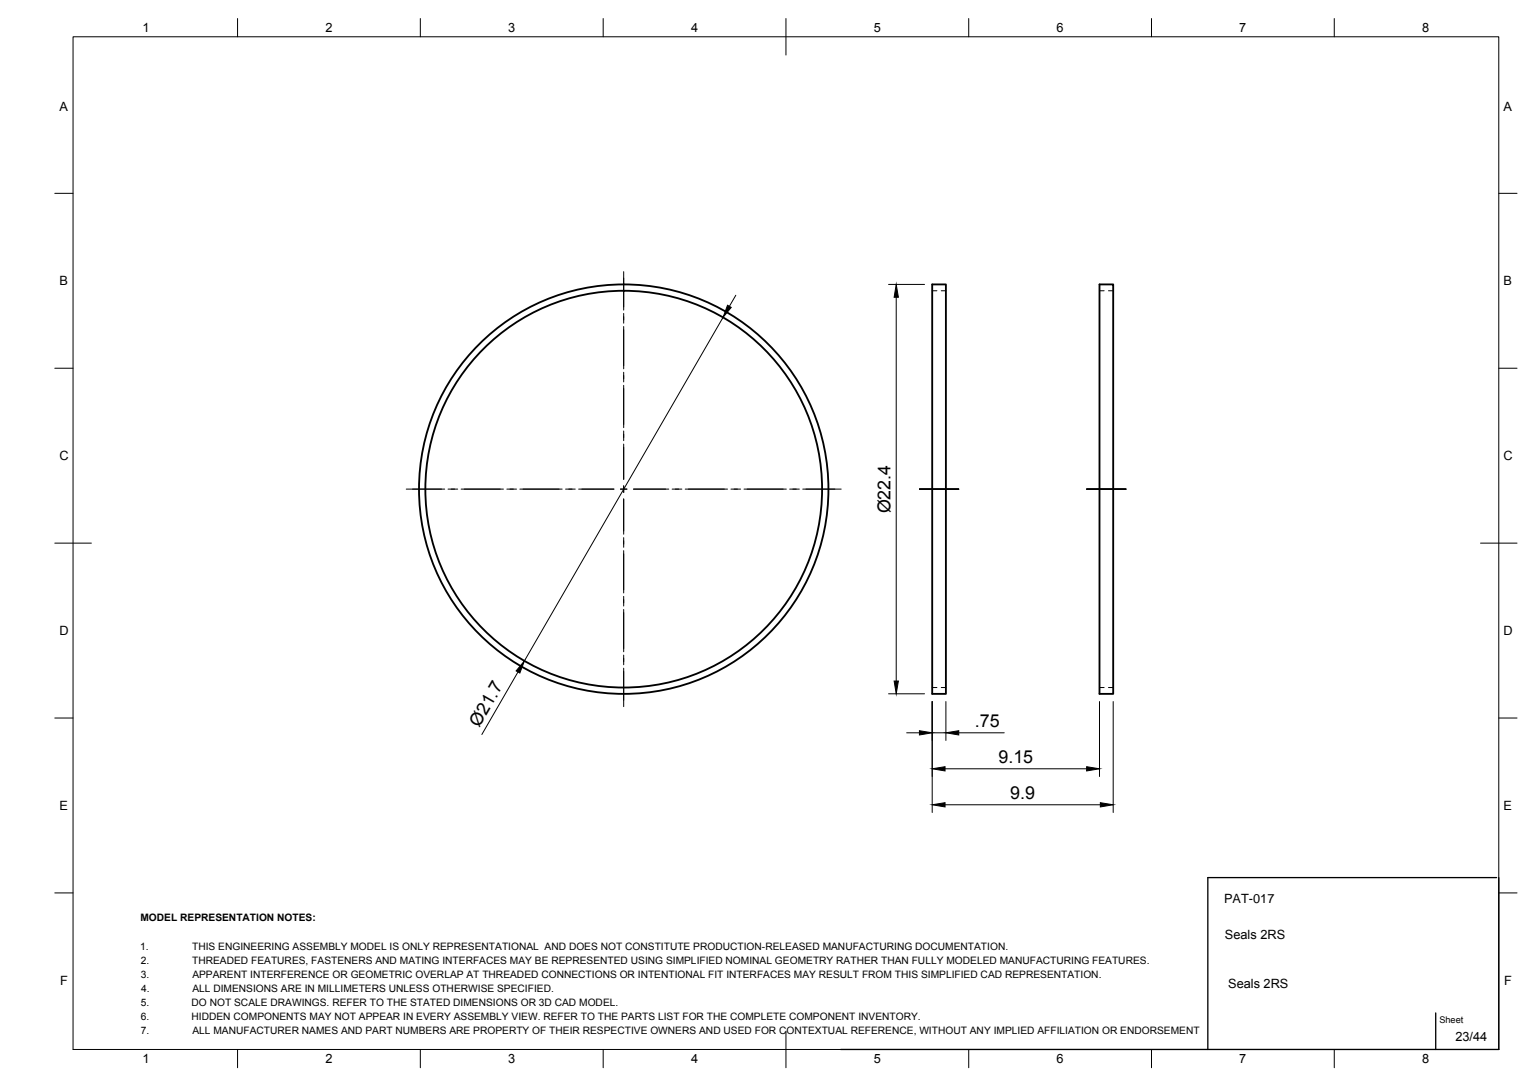
ISO-10303-21;
HEADER;
/* Generated by software containing ST-Developer
 * from STEP Tools, Inc. (www.steptools.com) 
 */

FILE_DESCRIPTION(
/* description */ ('Cam-and-follower valve demonstrator'),
/* implementation_level */ '2;1');

FILE_NAME(
/* name */ 'Seals 2RS.step',
/* time_stamp */ '2026-10-28T03:25:17-07:00',
/* author */ (''),
/* organization */ (''),
/* preprocessor_version */ 'ST-DEVELOPER v20.2',
/* originating_system */ 'Autodesk Translation Framework v15.17.0.0',
/* authorisation */ '');

FILE_SCHEMA (('AUTOMOTIVE_DESIGN { 1 0 10303 214 3 1 1 }'));
ENDSEC;

DATA;
#10=MECHANICAL_DESIGN_GEOMETRIC_PRESENTATION_REPRESENTATION('',(#434,#435),#12896);
#356=SHAPE_REPRESENTATION_RELATIONSHIP('SRR','None',#13073,#392);
#392=ADVANCED_BREP_SHAPE_REPRESENTATION('',(#477,#478),#12873);
#434=STYLED_ITEM('',(#13330),#477);
#435=STYLED_ITEM('',(#13330),#478);
#477=MANIFOLD_SOLID_BREP('Body1',#6201);
#478=MANIFOLD_SOLID_BREP('Body2',#6202);
#609=FACE_BOUND('',#1765,.T.);
#610=FACE_BOUND('',#1768,.T.);
#611=FACE_BOUND('',#1771,.T.);
#612=FACE_BOUND('',#1774,.T.);
#852=CIRCLE('',#7022,1.119765);
#853=CIRCLE('',#7023,1.085235);
#854=CIRCLE('',#7025,1.119765);
#855=CIRCLE('',#7027,1.085235);
#856=CIRCLE('',#7030,1.119765);
#857=CIRCLE('',#7031,1.085235);
#858=CIRCLE('',#7033,1.119765);
#859=CIRCLE('',#7035,1.085235);
#1046=CYLINDRICAL_SURFACE('',#7024,1.119765);
#1047=CYLINDRICAL_SURFACE('',#7028,1.085235);
#1048=CYLINDRICAL_SURFACE('',#7032,1.119765);
#1049=CYLINDRICAL_SURFACE('',#7036,1.085235);
#1282=FACE_OUTER_BOUND('',#1764,.T.);
#1283=FACE_OUTER_BOUND('',#1766,.T.);
#1284=FACE_OUTER_BOUND('',#1767,.T.);
#1285=FACE_OUTER_BOUND('',#1769,.T.);
#1286=FACE_OUTER_BOUND('',#1770,.T.);
#1287=FACE_OUTER_BOUND('',#1772,.T.);
#1288=FACE_OUTER_BOUND('',#1773,.T.);
#1289=FACE_OUTER_BOUND('',#1775,.T.);
#1764=EDGE_LOOP('',(#4929));
#1765=EDGE_LOOP('',(#4930));
#1766=EDGE_LOOP('',(#4931,#4932,#4933,#4934));
#1767=EDGE_LOOP('',(#4935));
#1768=EDGE_LOOP('',(#4936));
#1769=EDGE_LOOP('',(#4937,#4938,#4939,#4940));
#1770=EDGE_LOOP('',(#4941));
#1771=EDGE_LOOP('',(#4942));
#1772=EDGE_LOOP('',(#4943,#4944,#4945,#4946));
#1773=EDGE_LOOP('',(#4947));
#1774=EDGE_LOOP('',(#4948));
#1775=EDGE_LOOP('',(#4949,#4950,#4951,#4952));
#2204=LINE('',#11994,#2626);
#2205=LINE('',#11999,#2627);
#2206=LINE('',#12008,#2628);
#2207=LINE('',#12013,#2629);
#2626=VECTOR('',#8431,1.119765);
#2627=VECTOR('',#8438,1.085235);
#2628=VECTOR('',#8449,1.119765);
#2629=VECTOR('',#8456,1.085235);
#3125=VERTEX_POINT('',#11987);
#3126=VERTEX_POINT('',#11989);
#3127=VERTEX_POINT('',#11992);
#3128=VERTEX_POINT('',#11996);
#3129=VERTEX_POINT('',#12001);
#3130=VERTEX_POINT('',#12003);
#3131=VERTEX_POINT('',#12006);
#3132=VERTEX_POINT('',#12010);
#3761=EDGE_CURVE('',#3125,#3125,#852,.T.);
#3762=EDGE_CURVE('',#3126,#3126,#853,.T.);
#3763=EDGE_CURVE('',#3127,#3127,#854,.T.);
#3764=EDGE_CURVE('',#3127,#3125,#2204,.T.);
#3765=EDGE_CURVE('',#3128,#3128,#855,.T.);
#3766=EDGE_CURVE('',#3128,#3126,#2205,.T.);
#3767=EDGE_CURVE('',#3129,#3129,#856,.T.);
#3768=EDGE_CURVE('',#3130,#3130,#857,.T.);
#3769=EDGE_CURVE('',#3131,#3131,#858,.T.);
#3770=EDGE_CURVE('',#3131,#3129,#2206,.T.);
#3771=EDGE_CURVE('',#3132,#3132,#859,.T.);
#3772=EDGE_CURVE('',#3132,#3130,#2207,.T.);
#4929=ORIENTED_EDGE('',*,*,#3761,.F.);
#4930=ORIENTED_EDGE('',*,*,#3762,.T.);
#4931=ORIENTED_EDGE('',*,*,#3763,.F.);
#4932=ORIENTED_EDGE('',*,*,#3764,.T.);
#4933=ORIENTED_EDGE('',*,*,#3761,.T.);
#4934=ORIENTED_EDGE('',*,*,#3764,.F.);
#4935=ORIENTED_EDGE('',*,*,#3763,.T.);
#4936=ORIENTED_EDGE('',*,*,#3765,.F.);
#4937=ORIENTED_EDGE('',*,*,#3765,.T.);
#4938=ORIENTED_EDGE('',*,*,#3766,.T.);
#4939=ORIENTED_EDGE('',*,*,#3762,.F.);
#4940=ORIENTED_EDGE('',*,*,#3766,.F.);
#4941=ORIENTED_EDGE('',*,*,#3767,.F.);
#4942=ORIENTED_EDGE('',*,*,#3768,.T.);
#4943=ORIENTED_EDGE('',*,*,#3769,.F.);
#4944=ORIENTED_EDGE('',*,*,#3770,.T.);
#4945=ORIENTED_EDGE('',*,*,#3767,.T.);
#4946=ORIENTED_EDGE('',*,*,#3770,.F.);
#4947=ORIENTED_EDGE('',*,*,#3769,.T.);
#4948=ORIENTED_EDGE('',*,*,#3771,.F.);
#4949=ORIENTED_EDGE('',*,*,#3771,.T.);
#4950=ORIENTED_EDGE('',*,*,#3772,.T.);
#4951=ORIENTED_EDGE('',*,*,#3768,.F.);
#4952=ORIENTED_EDGE('',*,*,#3772,.F.);
#5690=PLANE('',#7021);
#5691=PLANE('',#7026);
#5692=PLANE('',#7029);
#5693=PLANE('',#7034);
#5998=ADVANCED_FACE('',(#1282,#609),#5690,.T.);
#5999=ADVANCED_FACE('',(#1283),#1046,.T.);
#6000=ADVANCED_FACE('',(#1284,#610),#5691,.T.);
#6001=ADVANCED_FACE('',(#1285),#1047,.F.);
#6002=ADVANCED_FACE('',(#1286,#611),#5692,.T.);
#6003=ADVANCED_FACE('',(#1287),#1048,.T.);
#6004=ADVANCED_FACE('',(#1288,#612),#5693,.T.);
#6005=ADVANCED_FACE('',(#1289),#1049,.F.);
#6201=CLOSED_SHELL('',(#5998,#5999,#6000,#6001));
#6202=CLOSED_SHELL('',(#6002,#6003,#6004,#6005));
#7020=AXIS2_PLACEMENT_3D('',#11985,#8419,#8420);
#7021=AXIS2_PLACEMENT_3D('',#11986,#8421,#8422);
#7022=AXIS2_PLACEMENT_3D('',#11988,#8423,#8424);
#7023=AXIS2_PLACEMENT_3D('',#11990,#8425,#8426);
#7024=AXIS2_PLACEMENT_3D('',#11991,#8427,#8428);
#7025=AXIS2_PLACEMENT_3D('',#11993,#8429,#8430);
#7026=AXIS2_PLACEMENT_3D('',#11995,#8432,#8433);
#7027=AXIS2_PLACEMENT_3D('',#11997,#8434,#8435);
#7028=AXIS2_PLACEMENT_3D('',#11998,#8436,#8437);
#7029=AXIS2_PLACEMENT_3D('',#12000,#8439,#8440);
#7030=AXIS2_PLACEMENT_3D('',#12002,#8441,#8442);
#7031=AXIS2_PLACEMENT_3D('',#12004,#8443,#8444);
#7032=AXIS2_PLACEMENT_3D('',#12005,#8445,#8446);
#7033=AXIS2_PLACEMENT_3D('',#12007,#8447,#8448);
#7034=AXIS2_PLACEMENT_3D('',#12009,#8450,#8451);
#7035=AXIS2_PLACEMENT_3D('',#12011,#8452,#8453);
#7036=AXIS2_PLACEMENT_3D('',#12012,#8454,#8455);
#8419=DIRECTION('axis',(0.,0.,1.));
#8420=DIRECTION('refdir',(1.,0.,0.));
#8421=DIRECTION('center_axis',(0.,1.,0.));
#8422=DIRECTION('ref_axis',(0.,0.,1.));
#8423=DIRECTION('center_axis',(0.,-1.,0.));
#8424=DIRECTION('ref_axis',(1.,0.,0.));
#8425=DIRECTION('center_axis',(0.,-1.,0.));
#8426=DIRECTION('ref_axis',(1.,0.,0.));
#8427=DIRECTION('center_axis',(0.,-1.,0.));
#8428=DIRECTION('ref_axis',(1.,0.,0.));
#8429=DIRECTION('center_axis',(0.,-1.,0.));
#8430=DIRECTION('ref_axis',(1.,0.,0.));
#8431=DIRECTION('',(0.,1.,0.));
#8432=DIRECTION('center_axis',(0.,-1.,0.));
#8433=DIRECTION('ref_axis',(0.,0.,-1.));
#8434=DIRECTION('center_axis',(0.,-1.,0.));
#8435=DIRECTION('ref_axis',(1.,0.,0.));
#8436=DIRECTION('center_axis',(0.,-1.,0.));
#8437=DIRECTION('ref_axis',(1.,0.,0.));
#8438=DIRECTION('',(0.,1.,0.));
#8439=DIRECTION('center_axis',(0.,1.,0.));
#8440=DIRECTION('ref_axis',(0.,0.,1.));
#8441=DIRECTION('center_axis',(0.,-1.,0.));
#8442=DIRECTION('ref_axis',(1.,0.,0.));
#8443=DIRECTION('center_axis',(0.,-1.,0.));
#8444=DIRECTION('ref_axis',(1.,0.,0.));
#8445=DIRECTION('center_axis',(0.,-1.,0.));
#8446=DIRECTION('ref_axis',(1.,0.,0.));
#8447=DIRECTION('center_axis',(0.,-1.,0.));
#8448=DIRECTION('ref_axis',(1.,0.,0.));
#8449=DIRECTION('',(0.,1.,0.));
#8450=DIRECTION('center_axis',(0.,-1.,0.));
#8451=DIRECTION('ref_axis',(0.,0.,-1.));
#8452=DIRECTION('center_axis',(0.,-1.,0.));
#8453=DIRECTION('ref_axis',(1.,0.,0.));
#8454=DIRECTION('center_axis',(0.,-1.,0.));
#8455=DIRECTION('ref_axis',(1.,0.,0.));
#8456=DIRECTION('',(0.,1.,0.));
#11985=CARTESIAN_POINT('',(0.,0.,0.));
#11986=CARTESIAN_POINT('Origin',(1.119765,0.495,0.));
#11987=CARTESIAN_POINT('',(-1.119765,0.495,-1.37131662304724E-16));
#11988=CARTESIAN_POINT('Origin',(0.,0.495,0.));
#11989=CARTESIAN_POINT('',(-1.085235,0.495,-1.32902956907268E-16));
#11990=CARTESIAN_POINT('Origin',(0.,0.495,0.));
#11991=CARTESIAN_POINT('Origin',(0.,0.4575,0.));
#11992=CARTESIAN_POINT('',(-1.119765,0.42,-1.37131662304724E-16));
#11993=CARTESIAN_POINT('Origin',(0.,0.42,0.));
#11994=CARTESIAN_POINT('',(-1.119765,0.4575,-1.37131662304724E-16));
#11995=CARTESIAN_POINT('Origin',(1.085235,0.42,0.));
#11996=CARTESIAN_POINT('',(-1.085235,0.42,-1.32902956907268E-16));
#11997=CARTESIAN_POINT('Origin',(0.,0.42,0.));
#11998=CARTESIAN_POINT('Origin',(0.,0.4575,0.));
#11999=CARTESIAN_POINT('',(-1.085235,0.4575,-1.32902956907268E-16));
#12000=CARTESIAN_POINT('Origin',(1.119765,-0.42,0.));
#12001=CARTESIAN_POINT('',(-1.119765,-0.42,-1.37131662304724E-16));
#12002=CARTESIAN_POINT('Origin',(0.,-0.42,0.));
#12003=CARTESIAN_POINT('',(-1.085235,-0.42,-1.32902956907268E-16));
#12004=CARTESIAN_POINT('Origin',(0.,-0.42,0.));
#12005=CARTESIAN_POINT('Origin',(0.,-0.4575,0.));
#12006=CARTESIAN_POINT('',(-1.119765,-0.495,-1.37131662304724E-16));
#12007=CARTESIAN_POINT('Origin',(0.,-0.495,0.));
#12008=CARTESIAN_POINT('',(-1.119765,-0.4575,-1.37131662304724E-16));
#12009=CARTESIAN_POINT('Origin',(1.085235,-0.495,0.));
#12010=CARTESIAN_POINT('',(-1.085235,-0.495,-1.32902956907268E-16));
#12011=CARTESIAN_POINT('Origin',(0.,-0.495,0.));
#12012=CARTESIAN_POINT('Origin',(0.,-0.4575,0.));
#12013=CARTESIAN_POINT('',(-1.085235,-0.4575,-1.32902956907268E-16));
#12830=UNCERTAINTY_MEASURE_WITH_UNIT(LENGTH_MEASURE(0.001),#12897,
'DISTANCE_ACCURACY_VALUE',
'Maximum model space distance between geometric entities at asserted c
onnectivities');
#12853=UNCERTAINTY_MEASURE_WITH_UNIT(LENGTH_MEASURE(0.001),#12897,
'DISTANCE_ACCURACY_VALUE',
'Maximum model space distance between geometric entities at asserted c
onnectivities');
#12873=(
GEOMETRIC_REPRESENTATION_CONTEXT(3)
GLOBAL_UNCERTAINTY_ASSIGNED_CONTEXT((#12830))
GLOBAL_UNIT_ASSIGNED_CONTEXT((#12897,#12899,#12900))
REPRESENTATION_CONTEXT('','3D')
);
#12896=(
GEOMETRIC_REPRESENTATION_CONTEXT(3)
GLOBAL_UNCERTAINTY_ASSIGNED_CONTEXT((#12853))
GLOBAL_UNIT_ASSIGNED_CONTEXT((#12897,#12899,#12900))
REPRESENTATION_CONTEXT('','3D')
);
#12897=(
LENGTH_UNIT()
NAMED_UNIT(*)
SI_UNIT(.CENTI.,.METRE.)
);
#12899=(
NAMED_UNIT(*)
PLANE_ANGLE_UNIT()
SI_UNIT($,.RADIAN.)
);
#12900=(
NAMED_UNIT(*)
SI_UNIT($,.STERADIAN.)
SOLID_ANGLE_UNIT()
);
#12920=SHAPE_DEFINITION_REPRESENTATION(#12962,#13073);
#12962=PRODUCT_DEFINITION_SHAPE('',$,#13116);
#13073=SHAPE_REPRESENTATION('',(#7020),#12873);
#13096=PRODUCT_DEFINITION_CONTEXT('part definition',#13224,'design');
#13116=PRODUCT_DEFINITION('Seals 2RS','Seals 2RS',#13158,#13096);
#13158=PRODUCT_DEFINITION_FORMATION('',$,#13245);
#13224=APPLICATION_CONTEXT(
'Core Data for Automotive Mechanical Design Process');
#13225=PRODUCT_CONTEXT('part definition',#13224,'mechanical');
#13245=PRODUCT('Seals 2RS','Seals 2RS','Seals 2RS',(#13225));
#13324=COLOUR_RGB('Grey',0.48,0.52,0.57);
#13325=FILL_AREA_STYLE_COLOUR('',#13324);
#13326=FILL_AREA_STYLE('',(#13325));
#13327=SURFACE_STYLE_FILL_AREA(#13326);
#13328=SURFACE_SIDE_STYLE('',(#13327));
#13329=SURFACE_STYLE_USAGE(.BOTH.,#13328);
#13330=PRESENTATION_STYLE_ASSIGNMENT((#13329));
ENDSEC;
END-ISO-10303-21;
